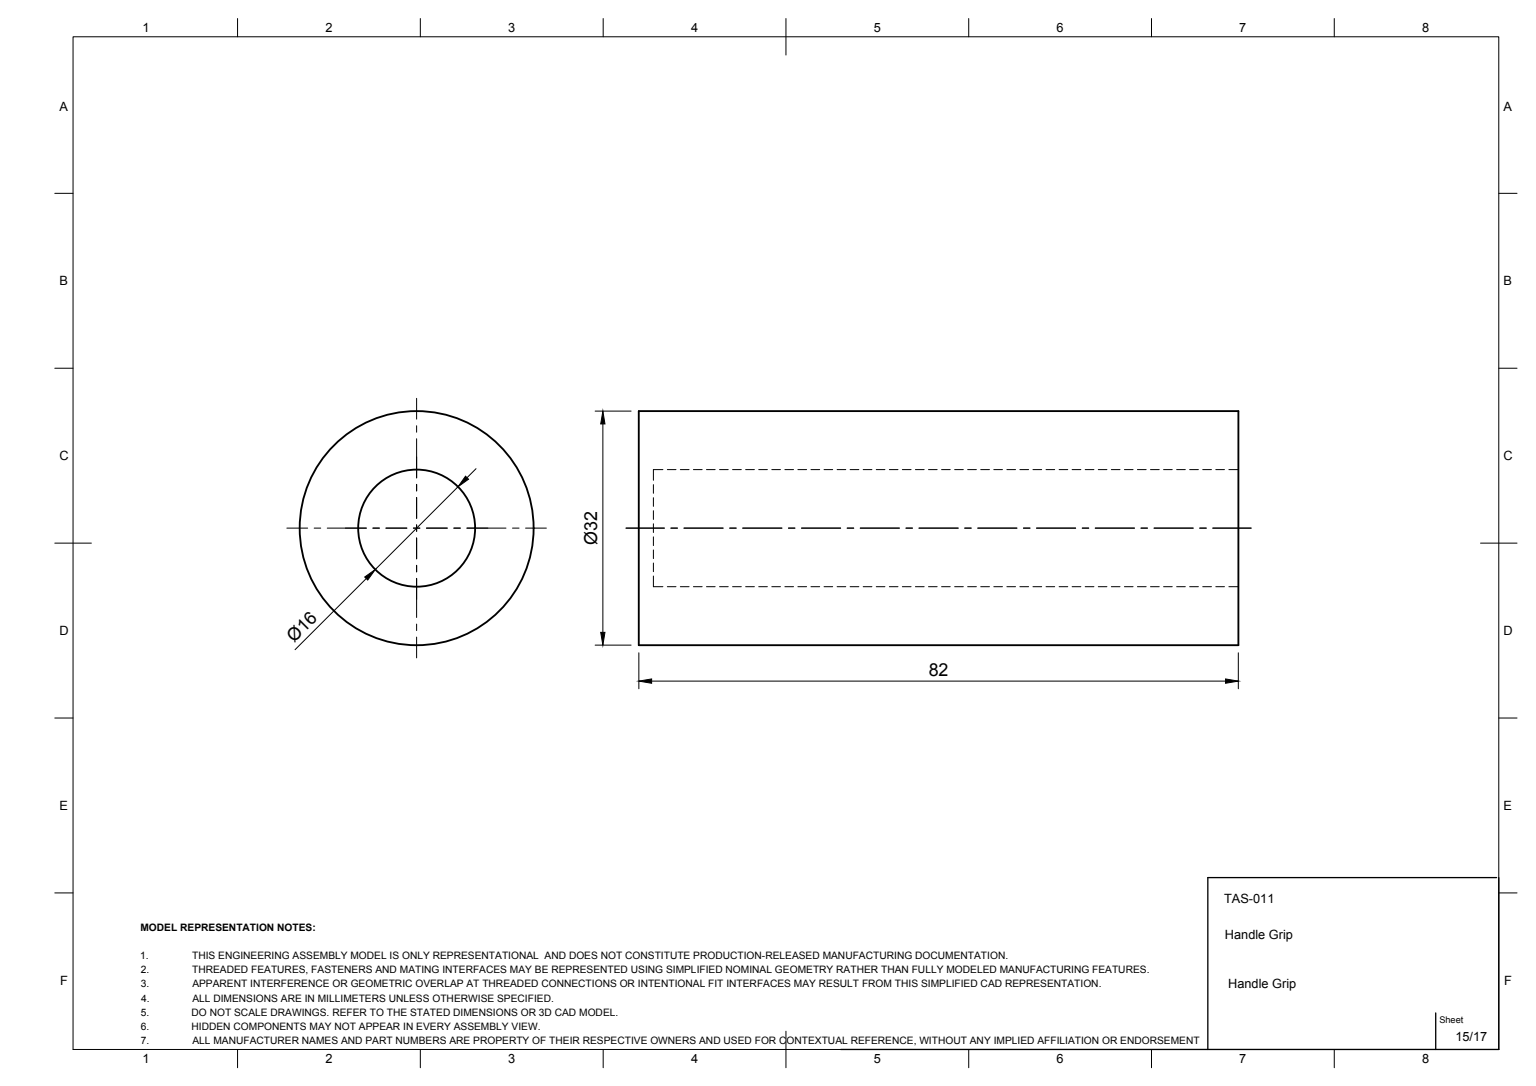
ISO-10303-21;
HEADER;
/* Generated by software containing ST-Developer
 * from STEP Tools, Inc. (www.steptools.com) 
 */

FILE_DESCRIPTION(
/* description */ (
'Independent manual bench leaf bending machine,200mm work width. Fabri
cated welded frame and folding leaf, repeated bushed and fully retaine
d hinge hardware, two handles with bonded grips, beveled clamping beam
 and modeledM12 clamp screws.2mm omitted-workpiece assembly reference 
gap, not a capacity claim. Native135deg hinge travel. Weld sizing, pro
duction fits, material condition, bending capacity, strength and life 
unassigned.'),
/* implementation_level */ '2;1');

FILE_NAME(
/* name */ 'Handle grip.step',
/* time_stamp */ '2026-11-14T09:11:34-08:00',
/* author */ (''),
/* organization */ (''),
/* preprocessor_version */ 'ST-DEVELOPER v20.2',
/* originating_system */ 'Autodesk Translation Framework v15.17.0.0',
/* authorisation */ '');

FILE_SCHEMA (('AUTOMOTIVE_DESIGN { 1 0 10303 214 3 1 1 }'));
ENDSEC;

DATA;
#10=MECHANICAL_DESIGN_GEOMETRIC_PRESENTATION_REPRESENTATION('',(#460),#37701);
#424=SHAPE_REPRESENTATION_RELATIONSHIP('SRR','None',#37793,#442);
#442=ADVANCED_BREP_SHAPE_REPRESENTATION('',(#478),#37697);
#460=STYLED_ITEM('',(#37882),#478);
#478=MANIFOLD_SOLID_BREP('Body1',#4158);
#510=FACE_BOUND('',#1035,.T.);
#588=PLANE('',#4626);
#589=PLANE('',#4628);
#590=PLANE('',#4634);
#790=FACE_OUTER_BOUND('',#1030,.T.);
#791=FACE_OUTER_BOUND('',#1031,.T.);
#792=FACE_OUTER_BOUND('',#1032,.T.);
#793=FACE_OUTER_BOUND('',#1033,.T.);
#794=FACE_OUTER_BOUND('',#1034,.T.);
#1030=EDGE_LOOP('',(#3739));
#1031=EDGE_LOOP('',(#3740));
#1032=EDGE_LOOP('',(#3741,#3742,#3743,#3744));
#1033=EDGE_LOOP('',(#3745,#3746,#3747,#3748));
#1034=EDGE_LOOP('',(#3749));
#1035=EDGE_LOOP('',(#3750));
#1293=LINE('',#37550,#1542);
#1294=LINE('',#37553,#1543);
#1542=VECTOR('',#5482,8.);
#1543=VECTOR('',#5485,16.);
#1617=CIRCLE('',#4627,8.);
#1618=CIRCLE('',#4629,16.);
#1619=CIRCLE('',#4631,8.);
#1620=CIRCLE('',#4633,16.);
#2029=VERTEX_POINT('',#37542);
#2030=VERTEX_POINT('',#37545);
#2031=VERTEX_POINT('',#37548);
#2032=VERTEX_POINT('',#37552);
#2603=EDGE_CURVE('',#2029,#2029,#1617,.T.);
#2604=EDGE_CURVE('',#2030,#2030,#1618,.F.);
#2605=EDGE_CURVE('',#2031,#2031,#1619,.T.);
#2606=EDGE_CURVE('',#2031,#2029,#1293,.T.);
#2607=EDGE_CURVE('',#2030,#2032,#1294,.T.);
#2608=EDGE_CURVE('',#2032,#2032,#1620,.F.);
#3739=ORIENTED_EDGE('',*,*,#2603,.T.);
#3740=ORIENTED_EDGE('',*,*,#2604,.T.);
#3741=ORIENTED_EDGE('',*,*,#2605,.T.);
#3742=ORIENTED_EDGE('',*,*,#2606,.T.);
#3743=ORIENTED_EDGE('',*,*,#2603,.F.);
#3744=ORIENTED_EDGE('',*,*,#2606,.F.);
#3745=ORIENTED_EDGE('',*,*,#2604,.F.);
#3746=ORIENTED_EDGE('',*,*,#2607,.T.);
#3747=ORIENTED_EDGE('',*,*,#2608,.T.);
#3748=ORIENTED_EDGE('',*,*,#2607,.F.);
#3749=ORIENTED_EDGE('',*,*,#2608,.F.);
#3750=ORIENTED_EDGE('',*,*,#2605,.F.);
#3922=CYLINDRICAL_SURFACE('',#4630,8.);
#3923=CYLINDRICAL_SURFACE('',#4632,16.);
#4120=ADVANCED_FACE('',(#790),#588,.F.);
#4121=ADVANCED_FACE('',(#791),#589,.T.);
#4122=ADVANCED_FACE('',(#792),#3922,.F.);
#4123=ADVANCED_FACE('',(#793),#3923,.T.);
#4124=ADVANCED_FACE('',(#794,#510),#590,.F.);
#4158=CLOSED_SHELL('',(#4120,#4121,#4122,#4123,#4124));
#4625=AXIS2_PLACEMENT_3D('',#37540,#5468,#5469);
#4626=AXIS2_PLACEMENT_3D('',#37541,#5470,#5471);
#4627=AXIS2_PLACEMENT_3D('',#37543,#5472,#5473);
#4628=AXIS2_PLACEMENT_3D('',#37544,#5474,#5475);
#4629=AXIS2_PLACEMENT_3D('',#37546,#5476,#5477);
#4630=AXIS2_PLACEMENT_3D('',#37547,#5478,#5479);
#4631=AXIS2_PLACEMENT_3D('',#37549,#5480,#5481);
#4632=AXIS2_PLACEMENT_3D('',#37551,#5483,#5484);
#4633=AXIS2_PLACEMENT_3D('',#37554,#5486,#5487);
#4634=AXIS2_PLACEMENT_3D('',#37555,#5488,#5489);
#5468=DIRECTION('axis',(0.,0.,1.));
#5469=DIRECTION('refdir',(1.,0.,0.));
#5470=DIRECTION('center_axis',(0.,0.,1.));
#5471=DIRECTION('ref_axis',(1.,0.,0.));
#5472=DIRECTION('center_axis',(0.,0.,-1.));
#5473=DIRECTION('ref_axis',(1.,0.,0.));
#5474=DIRECTION('center_axis',(0.,0.,1.));
#5475=DIRECTION('ref_axis',(1.,0.,0.));
#5476=DIRECTION('center_axis',(0.,0.,-1.));
#5477=DIRECTION('ref_axis',(1.,0.,0.));
#5478=DIRECTION('center_axis',(0.,0.,1.));
#5479=DIRECTION('ref_axis',(1.,0.,0.));
#5480=DIRECTION('center_axis',(0.,0.,-1.));
#5481=DIRECTION('ref_axis',(1.,0.,0.));
#5482=DIRECTION('',(0.,0.,1.));
#5483=DIRECTION('center_axis',(0.,0.,1.));
#5484=DIRECTION('ref_axis',(1.,0.,0.));
#5485=DIRECTION('',(0.,0.,-1.));
#5486=DIRECTION('center_axis',(0.,0.,-1.));
#5487=DIRECTION('ref_axis',(1.,0.,0.));
#5488=DIRECTION('center_axis',(0.,0.,1.));
#5489=DIRECTION('ref_axis',(1.,0.,0.));
#37540=CARTESIAN_POINT('',(0.,0.,0.));
#37541=CARTESIAN_POINT('Origin',(0.,0.,80.));
#37542=CARTESIAN_POINT('',(-8.,-9.79717439317883E-16,80.));
#37543=CARTESIAN_POINT('Origin',(0.,0.,80.));
#37544=CARTESIAN_POINT('Origin',(0.,0.,82.));
#37545=CARTESIAN_POINT('',(-16.,1.95943487863577E-15,82.));
#37546=CARTESIAN_POINT('Origin',(0.,0.,82.));
#37547=CARTESIAN_POINT('Origin',(0.,0.,0.));
#37548=CARTESIAN_POINT('',(-8.,-9.79717439317883E-16,0.));
#37549=CARTESIAN_POINT('Origin',(0.,0.,0.));
#37550=CARTESIAN_POINT('',(-8.,-9.79717439317883E-16,0.));
#37551=CARTESIAN_POINT('Origin',(0.,0.,0.));
#37552=CARTESIAN_POINT('',(-16.,1.95943487863577E-15,0.));
#37553=CARTESIAN_POINT('',(-16.,-1.95943487863577E-15,0.));
#37554=CARTESIAN_POINT('Origin',(0.,0.,0.));
#37555=CARTESIAN_POINT('Origin',(0.,0.,0.));
#37677=UNCERTAINTY_MEASURE_WITH_UNIT(LENGTH_MEASURE(0.01),#37702,
'DISTANCE_ACCURACY_VALUE',
'Maximum model space distance between geometric entities at asserted c
onnectivities');
#37681=UNCERTAINTY_MEASURE_WITH_UNIT(LENGTH_MEASURE(0.01),#37702,
'DISTANCE_ACCURACY_VALUE',
'Maximum model space distance between geometric entities at asserted c
onnectivities');
#37697=(
GEOMETRIC_REPRESENTATION_CONTEXT(3)
GLOBAL_UNCERTAINTY_ASSIGNED_CONTEXT((#37677))
GLOBAL_UNIT_ASSIGNED_CONTEXT((#37702,#37704,#37705))
REPRESENTATION_CONTEXT('','3D')
);
#37701=(
GEOMETRIC_REPRESENTATION_CONTEXT(3)
GLOBAL_UNCERTAINTY_ASSIGNED_CONTEXT((#37681))
GLOBAL_UNIT_ASSIGNED_CONTEXT((#37702,#37704,#37705))
REPRESENTATION_CONTEXT('','3D')
);
#37702=(
LENGTH_UNIT()
NAMED_UNIT(*)
SI_UNIT(.MILLI.,.METRE.)
);
#37704=(
NAMED_UNIT(*)
PLANE_ANGLE_UNIT()
SI_UNIT($,.RADIAN.)
);
#37705=(
NAMED_UNIT(*)
SI_UNIT($,.STERADIAN.)
SOLID_ANGLE_UNIT()
);
#37721=SHAPE_DEFINITION_REPRESENTATION(#37740,#37793);
#37740=PRODUCT_DEFINITION_SHAPE('',$,#37813);
#37793=SHAPE_REPRESENTATION('',(#4625),#37697);
#37797=PRODUCT_DEFINITION_CONTEXT('part definition',#37856,'design');
#37813=PRODUCT_DEFINITION('Handle Grip','Handle grip',#37832,#37797);
#37832=PRODUCT_DEFINITION_FORMATION('',$,#37873);
#37856=APPLICATION_CONTEXT(
'Core Data for Automotive Mechanical Design Process');
#37857=PRODUCT_CONTEXT('part definition',#37856,'mechanical');
#37873=PRODUCT('Handle Grip','Handle grip',$,(#37857));
#37882=PRESENTATION_STYLE_ASSIGNMENT((#37890));
#37890=SURFACE_STYLE_USAGE(.BOTH.,#37898);
#37898=SURFACE_SIDE_STYLE('',(#37906));
#37906=SURFACE_STYLE_FILL_AREA(#37914);
#37914=FILL_AREA_STYLE('Opaque(169,212,242)',(#37922));
#37922=FILL_AREA_STYLE_COLOUR('Opaque(169,212,242)',#37930);
#37930=COLOUR_RGB('Opaque(169,212,242)',0.662745098039216,0.831372549019608,
0.949019607843137);
ENDSEC;
END-ISO-10303-21;
